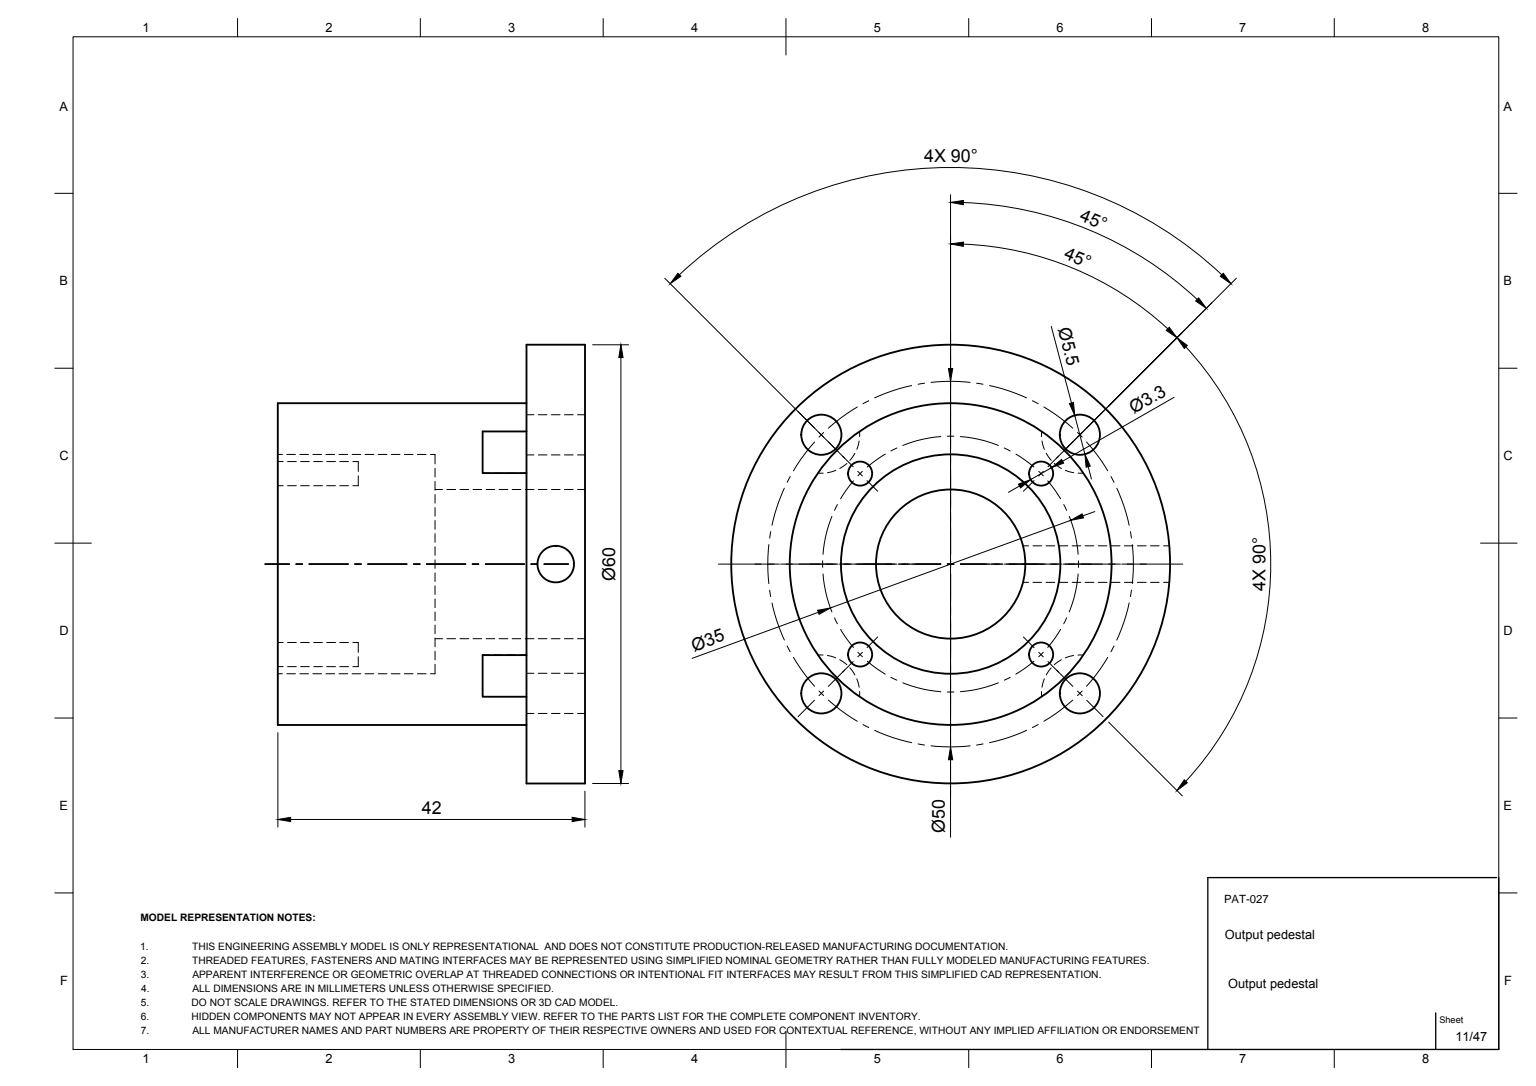
ISO-10303-21;
HEADER;
/* Generated by software containing ST-Developer
 * from STEP Tools, Inc. (www.steptools.com) 
 */

FILE_DESCRIPTION(
/* description */ ('Crank-driven oscillating fan base (mechanism only)'),

/* implementation_level */ '2;1');

FILE_NAME(
/* name */ 'Output pedestal.step',
/* time_stamp */ '2026-10-28T03:25:00-07:00',
/* author */ (''),
/* organization */ (''),
/* preprocessor_version */ 'ST-DEVELOPER v20.2',
/* originating_system */ 'Autodesk Translation Framework v15.17.0.0',
/* authorisation */ '');

FILE_SCHEMA (('AUTOMOTIVE_DESIGN { 1 0 10303 214 3 1 1 }'));
ENDSEC;

DATA;
#10=MECHANICAL_DESIGN_GEOMETRIC_PRESENTATION_REPRESENTATION('',(#443),#11916);
#320=B_SPLINE_CURVE_WITH_KNOTS('',3,(#9944,#9945,#9946,#9947,#9948,#9949,
#9950,#9951,#9952,#9953),.UNSPECIFIED.,.F.,.F.,(4,2,2,2,4),(0.,0.094594182476448,
0.189188364952896,0.283770357603024,0.378352350253152),.UNSPECIFIED.);
#321=B_SPLINE_CURVE_WITH_KNOTS('',3,(#9954,#9955,#9956,#9957,#9958,#9959,
#9960,#9961,#9962,#9963,#9964,#9965,#9966,#9967,#9968,#9969,#9970,#9971,
#9972,#9973,#9974,#9975,#9976,#9977,#9978,#9979),.UNSPECIFIED.,.F.,.F.,
(4,2,2,2,2,2,2,2,2,2,2,2,4),(0.378352350253152,0.47293434290328,0.567516335553408,
0.662110518029856,0.756704700506304,0.851298882982751,0.945893065459199,
1.04047505810933,1.13505705075946,1.22963904340958,1.32422103605971,1.41881521853616,
1.51340940101261),.UNSPECIFIED.);
#322=B_SPLINE_CURVE_WITH_KNOTS('',3,(#9983,#9984,#9985,#9986,#9987,#9988,
#9989,#9990,#9991,#9992,#9993,#9994,#9995,#9996,#9997,#9998,#9999,#10000,
#10001,#10002,#10003,#10004,#10005,#10006,#10007,#10008),.UNSPECIFIED.,
 .F.,.F.,(4,2,2,2,2,2,2,2,2,2,2,2,4),(0.,0.0942186410044058,0.188437282008812,
0.282655768798837,0.376874255588861,0.471092742378886,0.565311229168911,
0.659529870173317,0.753748511177723,0.847967152182129,0.942185793186535,
1.03640427997656,1.13062276676658),.UNSPECIFIED.);
#323=B_SPLINE_CURVE_WITH_KNOTS('',3,(#10009,#10010,#10011,#10012,#10013,
#10014,#10015,#10016,#10017,#10018),.UNSPECIFIED.,.F.,.F.,(4,2,2,2,4),(1.13062276676658,
1.22484125355661,1.31905974034663,1.41327838135104,1.50749702235545),
 .UNSPECIFIED.);
#363=SHAPE_REPRESENTATION_RELATIONSHIP('SRR','None',#12087,#403);
#403=ADVANCED_BREP_SHAPE_REPRESENTATION('',(#491),#11878);
#443=STYLED_ITEM('',(#12368),#491);
#491=MANIFOLD_SOLID_BREP('Body1',#6073);
#577=FACE_BOUND('',#1387,.T.);
#578=FACE_BOUND('',#1388,.T.);
#579=FACE_BOUND('',#1389,.T.);
#580=FACE_BOUND('',#1390,.T.);
#581=FACE_BOUND('',#1391,.T.);
#582=FACE_BOUND('',#1407,.T.);
#583=FACE_BOUND('',#1409,.T.);
#584=FACE_BOUND('',#1411,.T.);
#585=FACE_BOUND('',#1413,.T.);
#586=FACE_BOUND('',#1414,.T.);
#587=FACE_BOUND('',#1415,.T.);
#588=FACE_BOUND('',#1416,.T.);
#589=FACE_BOUND('',#1417,.T.);
#590=FACE_BOUND('',#1419,.T.);
#591=FACE_BOUND('',#1420,.T.);
#592=FACE_BOUND('',#1421,.T.);
#593=FACE_BOUND('',#1422,.T.);
#594=FACE_BOUND('',#1423,.T.);
#727=PLANE('',#6711);
#728=PLANE('',#6719);
#729=PLANE('',#6724);
#730=PLANE('',#6729);
#731=PLANE('',#6738);
#732=PLANE('',#6747);
#733=PLANE('',#6751);
#734=PLANE('',#6755);
#735=PLANE('',#6759);
#736=PLANE('',#6772);
#737=PLANE('',#6778);
#738=PLANE('',#6779);
#955=FACE_OUTER_BOUND('',#1377,.T.);
#956=FACE_OUTER_BOUND('',#1378,.T.);
#957=FACE_OUTER_BOUND('',#1379,.T.);
#958=FACE_OUTER_BOUND('',#1380,.T.);
#959=FACE_OUTER_BOUND('',#1381,.T.);
#960=FACE_OUTER_BOUND('',#1382,.T.);
#961=FACE_OUTER_BOUND('',#1383,.T.);
#962=FACE_OUTER_BOUND('',#1384,.T.);
#963=FACE_OUTER_BOUND('',#1385,.T.);
#964=FACE_OUTER_BOUND('',#1386,.T.);
#965=FACE_OUTER_BOUND('',#1392,.T.);
#966=FACE_OUTER_BOUND('',#1393,.T.);
#967=FACE_OUTER_BOUND('',#1394,.T.);
#968=FACE_OUTER_BOUND('',#1395,.T.);
#969=FACE_OUTER_BOUND('',#1396,.T.);
#970=FACE_OUTER_BOUND('',#1397,.T.);
#971=FACE_OUTER_BOUND('',#1398,.T.);
#972=FACE_OUTER_BOUND('',#1399,.T.);
#973=FACE_OUTER_BOUND('',#1400,.T.);
#974=FACE_OUTER_BOUND('',#1401,.T.);
#975=FACE_OUTER_BOUND('',#1402,.T.);
#976=FACE_OUTER_BOUND('',#1403,.T.);
#977=FACE_OUTER_BOUND('',#1404,.T.);
#978=FACE_OUTER_BOUND('',#1405,.T.);
#979=FACE_OUTER_BOUND('',#1406,.T.);
#980=FACE_OUTER_BOUND('',#1408,.T.);
#981=FACE_OUTER_BOUND('',#1410,.T.);
#982=FACE_OUTER_BOUND('',#1412,.T.);
#983=FACE_OUTER_BOUND('',#1418,.T.);
#1377=EDGE_LOOP('',(#4372,#4373));
#1378=EDGE_LOOP('',(#4374,#4375,#4376,#4377));
#1379=EDGE_LOOP('',(#4378,#4379,#4380,#4381));
#1380=EDGE_LOOP('',(#4382,#4383));
#1381=EDGE_LOOP('',(#4384,#4385,#4386,#4387));
#1382=EDGE_LOOP('',(#4388,#4389));
#1383=EDGE_LOOP('',(#4390,#4391,#4392,#4393));
#1384=EDGE_LOOP('',(#4394,#4395));
#1385=EDGE_LOOP('',(#4396,#4397,#4398,#4399,#4400,#4401,#4402,#4403,#4404,
#4405,#4406,#4407,#4408,#4409,#4410,#4411,#4412,#4413,#4414,#4415));
#1386=EDGE_LOOP('',(#4416));
#1387=EDGE_LOOP('',(#4417,#4418,#4419,#4420,#4421,#4422,#4423,#4424,#4425));
#1388=EDGE_LOOP('',(#4426));
#1389=EDGE_LOOP('',(#4427));
#1390=EDGE_LOOP('',(#4428));
#1391=EDGE_LOOP('',(#4429));
#1392=EDGE_LOOP('',(#4430,#4431,#4432,#4433));
#1393=EDGE_LOOP('',(#4434));
#1394=EDGE_LOOP('',(#4435,#4436,#4437,#4438));
#1395=EDGE_LOOP('',(#4439));
#1396=EDGE_LOOP('',(#4440,#4441,#4442,#4443));
#1397=EDGE_LOOP('',(#4444));
#1398=EDGE_LOOP('',(#4445,#4446,#4447,#4448));
#1399=EDGE_LOOP('',(#4449));
#1400=EDGE_LOOP('',(#4450,#4451,#4452,#4453,#4454,#4455));
#1401=EDGE_LOOP('',(#4456,#4457,#4458,#4459));
#1402=EDGE_LOOP('',(#4460,#4461,#4462,#4463));
#1403=EDGE_LOOP('',(#4464,#4465,#4466,#4467));
#1404=EDGE_LOOP('',(#4468,#4469,#4470,#4471));
#1405=EDGE_LOOP('',(#4472,#4473,#4474,#4475));
#1406=EDGE_LOOP('',(#4476));
#1407=EDGE_LOOP('',(#4477));
#1408=EDGE_LOOP('',(#4478,#4479,#4480,#4481));
#1409=EDGE_LOOP('',(#4482,#4483));
#1410=EDGE_LOOP('',(#4484,#4485,#4486,#4487));
#1411=EDGE_LOOP('',(#4488,#4489));
#1412=EDGE_LOOP('',(#4490));
#1413=EDGE_LOOP('',(#4491));
#1414=EDGE_LOOP('',(#4492));
#1415=EDGE_LOOP('',(#4493));
#1416=EDGE_LOOP('',(#4494));
#1417=EDGE_LOOP('',(#4495));
#1418=EDGE_LOOP('',(#4496));
#1419=EDGE_LOOP('',(#4497));
#1420=EDGE_LOOP('',(#4498));
#1421=EDGE_LOOP('',(#4499));
#1422=EDGE_LOOP('',(#4500));
#1423=EDGE_LOOP('',(#4501));
#1872=LINE('',#9855,#2205);
#1873=LINE('',#9858,#2206);
#1874=LINE('',#9862,#2207);
#1875=LINE('',#9866,#2208);
#1876=LINE('',#9873,#2209);
#1877=LINE('',#9877,#2210);
#1878=LINE('',#9884,#2211);
#1879=LINE('',#9888,#2212);
#1880=LINE('',#9896,#2213);
#1881=LINE('',#9917,#2214);
#1882=LINE('',#9924,#2215);
#1883=LINE('',#9931,#2216);
#1884=LINE('',#9938,#2217);
#1885=LINE('',#9981,#2218);
#1886=LINE('',#10022,#2219);
#1887=LINE('',#10026,#2220);
#1888=LINE('',#10030,#2221);
#1889=LINE('',#10034,#2222);
#1890=LINE('',#10039,#2223);
#1891=LINE('',#10046,#2224);
#1892=LINE('',#10050,#2225);
#2205=VECTOR('',#7797,1.);
#2206=VECTOR('',#7800,1.);
#2207=VECTOR('',#7803,1.);
#2208=VECTOR('',#7806,1.);
#2209=VECTOR('',#7815,1.);
#2210=VECTOR('',#7818,1.);
#2211=VECTOR('',#7827,1.);
#2212=VECTOR('',#7830,1.);
#2213=VECTOR('',#7841,2.2);
#2214=VECTOR('',#7868,0.165);
#2215=VECTOR('',#7877,0.165);
#2216=VECTOR('',#7886,0.164999999999999);
#2217=VECTOR('',#7895,0.164999999999999);
#2218=VECTOR('',#7902,0.25);
#2219=VECTOR('',#7907,0.275);
#2220=VECTOR('',#7912,0.275);
#2221=VECTOR('',#7917,0.275);
#2222=VECTOR('',#7922,0.275);
#2223=VECTOR('',#7927,1.5);
#2224=VECTOR('',#7936,3.);
#2225=VECTOR('',#7941,1.02);
#2538=CIRCLE('',#6712,2.2);
#2539=CIRCLE('',#6713,0.525);
#2540=CIRCLE('',#6715,0.525);
#2541=CIRCLE('',#6717,0.525);
#2542=CIRCLE('',#6718,0.525);
#2543=CIRCLE('',#6720,2.2);
#2544=CIRCLE('',#6722,0.525);
#2545=CIRCLE('',#6723,0.525);
#2546=CIRCLE('',#6725,2.2);
#2547=CIRCLE('',#6727,0.525);
#2548=CIRCLE('',#6728,0.525);
#2549=CIRCLE('',#6730,2.2);
#2550=CIRCLE('',#6732,2.2);
#2551=CIRCLE('',#6733,2.2);
#2552=CIRCLE('',#6734,2.2);
#2553=CIRCLE('',#6735,2.2);
#2554=CIRCLE('',#6736,2.2);
#2555=CIRCLE('',#6737,2.2);
#2556=CIRCLE('',#6739,3.);
#2557=CIRCLE('',#6740,0.275);
#2558=CIRCLE('',#6741,0.275);
#2559=CIRCLE('',#6742,0.275);
#2560=CIRCLE('',#6743,0.275);
#2561=CIRCLE('',#6745,0.165);
#2562=CIRCLE('',#6746,0.165);
#2563=CIRCLE('',#6749,0.165);
#2564=CIRCLE('',#6750,0.165);
#2565=CIRCLE('',#6753,0.164999999999999);
#2566=CIRCLE('',#6754,0.164999999999999);
#2567=CIRCLE('',#6757,0.164999999999999);
#2568=CIRCLE('',#6758,0.164999999999999);
#2569=CIRCLE('',#6762,0.275);
#2570=CIRCLE('',#6764,0.275);
#2571=CIRCLE('',#6766,0.275);
#2572=CIRCLE('',#6768,0.275);
#2573=CIRCLE('',#6770,1.5);
#2574=CIRCLE('',#6771,1.5);
#2575=CIRCLE('',#6773,1.02);
#2576=CIRCLE('',#6775,3.);
#2577=CIRCLE('',#6777,1.02);
#2931=VERTEX_POINT('',#9849);
#2932=VERTEX_POINT('',#9850);
#2933=VERTEX_POINT('',#9854);
#2934=VERTEX_POINT('',#9856);
#2935=VERTEX_POINT('',#9860);
#2936=VERTEX_POINT('',#9861);
#2937=VERTEX_POINT('',#9863);
#2938=VERTEX_POINT('',#9865);
#2939=VERTEX_POINT('',#9871);
#2940=VERTEX_POINT('',#9872);
#2941=VERTEX_POINT('',#9874);
#2942=VERTEX_POINT('',#9876);
#2943=VERTEX_POINT('',#9882);
#2944=VERTEX_POINT('',#9883);
#2945=VERTEX_POINT('',#9885);
#2946=VERTEX_POINT('',#9887);
#2947=VERTEX_POINT('',#9893);
#2948=VERTEX_POINT('',#9895);
#2949=VERTEX_POINT('',#9903);
#2950=VERTEX_POINT('',#9905);
#2951=VERTEX_POINT('',#9907);
#2952=VERTEX_POINT('',#9909);
#2953=VERTEX_POINT('',#9911);
#2954=VERTEX_POINT('',#9914);
#2955=VERTEX_POINT('',#9916);
#2956=VERTEX_POINT('',#9921);
#2957=VERTEX_POINT('',#9923);
#2958=VERTEX_POINT('',#9928);
#2959=VERTEX_POINT('',#9930);
#2960=VERTEX_POINT('',#9935);
#2961=VERTEX_POINT('',#9937);
#2962=VERTEX_POINT('',#9942);
#2963=VERTEX_POINT('',#9943);
#2964=VERTEX_POINT('',#9980);
#2965=VERTEX_POINT('',#9982);
#2966=VERTEX_POINT('',#10020);
#2967=VERTEX_POINT('',#10024);
#2968=VERTEX_POINT('',#10028);
#2969=VERTEX_POINT('',#10032);
#2970=VERTEX_POINT('',#10036);
#2971=VERTEX_POINT('',#10038);
#2972=VERTEX_POINT('',#10042);
#2973=VERTEX_POINT('',#10045);
#2974=VERTEX_POINT('',#10049);
#3481=EDGE_CURVE('',#2931,#2932,#2538,.T.);
#3482=EDGE_CURVE('',#2932,#2931,#2539,.T.);
#3483=EDGE_CURVE('',#2933,#2931,#1872,.T.);
#3484=EDGE_CURVE('',#2934,#2933,#2540,.T.);
#3485=EDGE_CURVE('',#2932,#2934,#1873,.T.);
#3486=EDGE_CURVE('',#2935,#2936,#1874,.T.);
#3487=EDGE_CURVE('',#2935,#2937,#2541,.T.);
#3488=EDGE_CURVE('',#2938,#2937,#1875,.T.);
#3489=EDGE_CURVE('',#2936,#2938,#2542,.T.);
#3490=EDGE_CURVE('',#2937,#2935,#2543,.T.);
#3491=EDGE_CURVE('',#2939,#2940,#1876,.T.);
#3492=EDGE_CURVE('',#2939,#2941,#2544,.T.);
#3493=EDGE_CURVE('',#2942,#2941,#1877,.T.);
#3494=EDGE_CURVE('',#2940,#2942,#2545,.T.);
#3495=EDGE_CURVE('',#2941,#2939,#2546,.T.);
#3496=EDGE_CURVE('',#2943,#2944,#1878,.T.);
#3497=EDGE_CURVE('',#2943,#2945,#2547,.T.);
#3498=EDGE_CURVE('',#2946,#2945,#1879,.T.);
#3499=EDGE_CURVE('',#2944,#2946,#2548,.T.);
#3500=EDGE_CURVE('',#2945,#2943,#2549,.T.);
#3501=EDGE_CURVE('',#2947,#2947,#2550,.T.);
#3502=EDGE_CURVE('',#2947,#2948,#1880,.T.);
#3503=EDGE_CURVE('',#2948,#2933,#2551,.T.);
#3504=EDGE_CURVE('',#2934,#2946,#2552,.T.);
#3505=EDGE_CURVE('',#2944,#2942,#2553,.T.);
#3506=EDGE_CURVE('',#2940,#2938,#2554,.T.);
#3507=EDGE_CURVE('',#2936,#2948,#2555,.T.);
#3508=EDGE_CURVE('',#2949,#2949,#2556,.T.);
#3509=EDGE_CURVE('',#2950,#2950,#2557,.T.);
#3510=EDGE_CURVE('',#2951,#2951,#2558,.T.);
#3511=EDGE_CURVE('',#2952,#2952,#2559,.T.);
#3512=EDGE_CURVE('',#2953,#2953,#2560,.T.);
#3513=EDGE_CURVE('',#2954,#2954,#2561,.T.);
#3514=EDGE_CURVE('',#2954,#2955,#1881,.T.);
#3515=EDGE_CURVE('',#2955,#2955,#2562,.T.);
#3516=EDGE_CURVE('',#2956,#2956,#2563,.T.);
#3517=EDGE_CURVE('',#2956,#2957,#1882,.T.);
#3518=EDGE_CURVE('',#2957,#2957,#2564,.T.);
#3519=EDGE_CURVE('',#2958,#2958,#2565,.T.);
#3520=EDGE_CURVE('',#2958,#2959,#1883,.T.);
#3521=EDGE_CURVE('',#2959,#2959,#2566,.T.);
#3522=EDGE_CURVE('',#2960,#2960,#2567,.T.);
#3523=EDGE_CURVE('',#2960,#2961,#1884,.T.);
#3524=EDGE_CURVE('',#2961,#2961,#2568,.T.);
#3525=EDGE_CURVE('',#2962,#2963,#320,.T.);
#3526=EDGE_CURVE('',#2963,#2962,#321,.T.);
#3527=EDGE_CURVE('',#2963,#2964,#1885,.T.);
#3528=EDGE_CURVE('',#2965,#2964,#322,.T.);
#3529=EDGE_CURVE('',#2964,#2965,#323,.T.);
#3530=EDGE_CURVE('',#2966,#2966,#2569,.T.);
#3531=EDGE_CURVE('',#2966,#2950,#1886,.T.);
#3532=EDGE_CURVE('',#2967,#2967,#2570,.T.);
#3533=EDGE_CURVE('',#2967,#2953,#1887,.T.);
#3534=EDGE_CURVE('',#2968,#2968,#2571,.T.);
#3535=EDGE_CURVE('',#2968,#2951,#1888,.T.);
#3536=EDGE_CURVE('',#2969,#2969,#2572,.T.);
#3537=EDGE_CURVE('',#2969,#2952,#1889,.T.);
#3538=EDGE_CURVE('',#2970,#2970,#2573,.T.);
#3539=EDGE_CURVE('',#2970,#2971,#1890,.T.);
#3540=EDGE_CURVE('',#2971,#2971,#2574,.T.);
#3541=EDGE_CURVE('',#2972,#2972,#2575,.T.);
#3542=EDGE_CURVE('',#2949,#2973,#1891,.T.);
#3543=EDGE_CURVE('',#2973,#2973,#2576,.T.);
#3544=EDGE_CURVE('',#2972,#2974,#1892,.T.);
#3545=EDGE_CURVE('',#2974,#2974,#2577,.T.);
#4372=ORIENTED_EDGE('',*,*,#3481,.F.);
#4373=ORIENTED_EDGE('',*,*,#3482,.F.);
#4374=ORIENTED_EDGE('',*,*,#3483,.F.);
#4375=ORIENTED_EDGE('',*,*,#3484,.F.);
#4376=ORIENTED_EDGE('',*,*,#3485,.F.);
#4377=ORIENTED_EDGE('',*,*,#3482,.T.);
#4378=ORIENTED_EDGE('',*,*,#3486,.F.);
#4379=ORIENTED_EDGE('',*,*,#3487,.T.);
#4380=ORIENTED_EDGE('',*,*,#3488,.F.);
#4381=ORIENTED_EDGE('',*,*,#3489,.F.);
#4382=ORIENTED_EDGE('',*,*,#3490,.F.);
#4383=ORIENTED_EDGE('',*,*,#3487,.F.);
#4384=ORIENTED_EDGE('',*,*,#3491,.F.);
#4385=ORIENTED_EDGE('',*,*,#3492,.T.);
#4386=ORIENTED_EDGE('',*,*,#3493,.F.);
#4387=ORIENTED_EDGE('',*,*,#3494,.F.);
#4388=ORIENTED_EDGE('',*,*,#3495,.F.);
#4389=ORIENTED_EDGE('',*,*,#3492,.F.);
#4390=ORIENTED_EDGE('',*,*,#3496,.F.);
#4391=ORIENTED_EDGE('',*,*,#3497,.T.);
#4392=ORIENTED_EDGE('',*,*,#3498,.F.);
#4393=ORIENTED_EDGE('',*,*,#3499,.F.);
#4394=ORIENTED_EDGE('',*,*,#3500,.F.);
#4395=ORIENTED_EDGE('',*,*,#3497,.F.);
#4396=ORIENTED_EDGE('',*,*,#3501,.F.);
#4397=ORIENTED_EDGE('',*,*,#3502,.T.);
#4398=ORIENTED_EDGE('',*,*,#3503,.T.);
#4399=ORIENTED_EDGE('',*,*,#3483,.T.);
#4400=ORIENTED_EDGE('',*,*,#3481,.T.);
#4401=ORIENTED_EDGE('',*,*,#3485,.T.);
#4402=ORIENTED_EDGE('',*,*,#3504,.T.);
#4403=ORIENTED_EDGE('',*,*,#3498,.T.);
#4404=ORIENTED_EDGE('',*,*,#3500,.T.);
#4405=ORIENTED_EDGE('',*,*,#3496,.T.);
#4406=ORIENTED_EDGE('',*,*,#3505,.T.);
#4407=ORIENTED_EDGE('',*,*,#3493,.T.);
#4408=ORIENTED_EDGE('',*,*,#3495,.T.);
#4409=ORIENTED_EDGE('',*,*,#3491,.T.);
#4410=ORIENTED_EDGE('',*,*,#3506,.T.);
#4411=ORIENTED_EDGE('',*,*,#3488,.T.);
#4412=ORIENTED_EDGE('',*,*,#3490,.T.);
#4413=ORIENTED_EDGE('',*,*,#3486,.T.);
#4414=ORIENTED_EDGE('',*,*,#3507,.T.);
#4415=ORIENTED_EDGE('',*,*,#3502,.F.);
#4416=ORIENTED_EDGE('',*,*,#3508,.T.);
#4417=ORIENTED_EDGE('',*,*,#3507,.F.);
#4418=ORIENTED_EDGE('',*,*,#3489,.T.);
#4419=ORIENTED_EDGE('',*,*,#3506,.F.);
#4420=ORIENTED_EDGE('',*,*,#3494,.T.);
#4421=ORIENTED_EDGE('',*,*,#3505,.F.);
#4422=ORIENTED_EDGE('',*,*,#3499,.T.);
#4423=ORIENTED_EDGE('',*,*,#3504,.F.);
#4424=ORIENTED_EDGE('',*,*,#3484,.T.);
#4425=ORIENTED_EDGE('',*,*,#3503,.F.);
#4426=ORIENTED_EDGE('',*,*,#3509,.T.);
#4427=ORIENTED_EDGE('',*,*,#3510,.T.);
#4428=ORIENTED_EDGE('',*,*,#3511,.T.);
#4429=ORIENTED_EDGE('',*,*,#3512,.T.);
#4430=ORIENTED_EDGE('',*,*,#3513,.F.);
#4431=ORIENTED_EDGE('',*,*,#3514,.T.);
#4432=ORIENTED_EDGE('',*,*,#3515,.F.);
#4433=ORIENTED_EDGE('',*,*,#3514,.F.);
#4434=ORIENTED_EDGE('',*,*,#3513,.T.);
#4435=ORIENTED_EDGE('',*,*,#3516,.F.);
#4436=ORIENTED_EDGE('',*,*,#3517,.T.);
#4437=ORIENTED_EDGE('',*,*,#3518,.F.);
#4438=ORIENTED_EDGE('',*,*,#3517,.F.);
#4439=ORIENTED_EDGE('',*,*,#3516,.T.);
#4440=ORIENTED_EDGE('',*,*,#3519,.F.);
#4441=ORIENTED_EDGE('',*,*,#3520,.T.);
#4442=ORIENTED_EDGE('',*,*,#3521,.F.);
#4443=ORIENTED_EDGE('',*,*,#3520,.F.);
#4444=ORIENTED_EDGE('',*,*,#3519,.T.);
#4445=ORIENTED_EDGE('',*,*,#3522,.F.);
#4446=ORIENTED_EDGE('',*,*,#3523,.T.);
#4447=ORIENTED_EDGE('',*,*,#3524,.F.);
#4448=ORIENTED_EDGE('',*,*,#3523,.F.);
#4449=ORIENTED_EDGE('',*,*,#3522,.T.);
#4450=ORIENTED_EDGE('',*,*,#3525,.F.);
#4451=ORIENTED_EDGE('',*,*,#3526,.F.);
#4452=ORIENTED_EDGE('',*,*,#3527,.T.);
#4453=ORIENTED_EDGE('',*,*,#3528,.F.);
#4454=ORIENTED_EDGE('',*,*,#3529,.F.);
#4455=ORIENTED_EDGE('',*,*,#3527,.F.);
#4456=ORIENTED_EDGE('',*,*,#3530,.F.);
#4457=ORIENTED_EDGE('',*,*,#3531,.T.);
#4458=ORIENTED_EDGE('',*,*,#3509,.F.);
#4459=ORIENTED_EDGE('',*,*,#3531,.F.);
#4460=ORIENTED_EDGE('',*,*,#3532,.F.);
#4461=ORIENTED_EDGE('',*,*,#3533,.T.);
#4462=ORIENTED_EDGE('',*,*,#3512,.F.);
#4463=ORIENTED_EDGE('',*,*,#3533,.F.);
#4464=ORIENTED_EDGE('',*,*,#3534,.F.);
#4465=ORIENTED_EDGE('',*,*,#3535,.T.);
#4466=ORIENTED_EDGE('',*,*,#3510,.F.);
#4467=ORIENTED_EDGE('',*,*,#3535,.F.);
#4468=ORIENTED_EDGE('',*,*,#3536,.F.);
#4469=ORIENTED_EDGE('',*,*,#3537,.T.);
#4470=ORIENTED_EDGE('',*,*,#3511,.F.);
#4471=ORIENTED_EDGE('',*,*,#3537,.F.);
#4472=ORIENTED_EDGE('',*,*,#3538,.F.);
#4473=ORIENTED_EDGE('',*,*,#3539,.T.);
#4474=ORIENTED_EDGE('',*,*,#3540,.F.);
#4475=ORIENTED_EDGE('',*,*,#3539,.F.);
#4476=ORIENTED_EDGE('',*,*,#3538,.T.);
#4477=ORIENTED_EDGE('',*,*,#3541,.F.);
#4478=ORIENTED_EDGE('',*,*,#3508,.F.);
#4479=ORIENTED_EDGE('',*,*,#3542,.T.);
#4480=ORIENTED_EDGE('',*,*,#3543,.T.);
#4481=ORIENTED_EDGE('',*,*,#3542,.F.);
#4482=ORIENTED_EDGE('',*,*,#3528,.T.);
#4483=ORIENTED_EDGE('',*,*,#3529,.T.);
#4484=ORIENTED_EDGE('',*,*,#3541,.T.);
#4485=ORIENTED_EDGE('',*,*,#3544,.T.);
#4486=ORIENTED_EDGE('',*,*,#3545,.T.);
#4487=ORIENTED_EDGE('',*,*,#3544,.F.);
#4488=ORIENTED_EDGE('',*,*,#3525,.T.);
#4489=ORIENTED_EDGE('',*,*,#3526,.T.);
#4490=ORIENTED_EDGE('',*,*,#3501,.T.);
#4491=ORIENTED_EDGE('',*,*,#3540,.T.);
#4492=ORIENTED_EDGE('',*,*,#3524,.T.);
#4493=ORIENTED_EDGE('',*,*,#3521,.T.);
#4494=ORIENTED_EDGE('',*,*,#3518,.T.);
#4495=ORIENTED_EDGE('',*,*,#3515,.T.);
#4496=ORIENTED_EDGE('',*,*,#3543,.F.);
#4497=ORIENTED_EDGE('',*,*,#3545,.F.);
#4498=ORIENTED_EDGE('',*,*,#3536,.T.);
#4499=ORIENTED_EDGE('',*,*,#3534,.T.);
#4500=ORIENTED_EDGE('',*,*,#3532,.T.);
#4501=ORIENTED_EDGE('',*,*,#3530,.T.);
#5580=CYLINDRICAL_SURFACE('',#6714,0.525);
#5581=CYLINDRICAL_SURFACE('',#6716,0.525);
#5582=CYLINDRICAL_SURFACE('',#6721,0.525);
#5583=CYLINDRICAL_SURFACE('',#6726,0.525);
#5584=CYLINDRICAL_SURFACE('',#6731,2.2);
#5585=CYLINDRICAL_SURFACE('',#6744,0.165);
#5586=CYLINDRICAL_SURFACE('',#6748,0.165);
#5587=CYLINDRICAL_SURFACE('',#6752,0.164999999999999);
#5588=CYLINDRICAL_SURFACE('',#6756,0.164999999999999);
#5589=CYLINDRICAL_SURFACE('',#6760,0.25);
#5590=CYLINDRICAL_SURFACE('',#6761,0.275);
#5591=CYLINDRICAL_SURFACE('',#6763,0.275);
#5592=CYLINDRICAL_SURFACE('',#6765,0.275);
#5593=CYLINDRICAL_SURFACE('',#6767,0.275);
#5594=CYLINDRICAL_SURFACE('',#6769,1.5);
#5595=CYLINDRICAL_SURFACE('',#6774,3.);
#5596=CYLINDRICAL_SURFACE('',#6776,1.02);
#5761=ADVANCED_FACE('',(#955),#727,.F.);
#5762=ADVANCED_FACE('',(#956),#5580,.F.);
#5763=ADVANCED_FACE('',(#957),#5581,.F.);
#5764=ADVANCED_FACE('',(#958),#728,.F.);
#5765=ADVANCED_FACE('',(#959),#5582,.F.);
#5766=ADVANCED_FACE('',(#960),#729,.F.);
#5767=ADVANCED_FACE('',(#961),#5583,.F.);
#5768=ADVANCED_FACE('',(#962),#730,.F.);
#5769=ADVANCED_FACE('',(#963),#5584,.T.);
#5770=ADVANCED_FACE('',(#964,#577,#578,#579,#580,#581),#731,.T.);
#5771=ADVANCED_FACE('',(#965),#5585,.F.);
#5772=ADVANCED_FACE('',(#966),#732,.T.);
#5773=ADVANCED_FACE('',(#967),#5586,.F.);
#5774=ADVANCED_FACE('',(#968),#733,.T.);
#5775=ADVANCED_FACE('',(#969),#5587,.F.);
#5776=ADVANCED_FACE('',(#970),#734,.T.);
#5777=ADVANCED_FACE('',(#971),#5588,.F.);
#5778=ADVANCED_FACE('',(#972),#735,.T.);
#5779=ADVANCED_FACE('',(#973),#5589,.F.);
#5780=ADVANCED_FACE('',(#974),#5590,.F.);
#5781=ADVANCED_FACE('',(#975),#5591,.F.);
#5782=ADVANCED_FACE('',(#976),#5592,.F.);
#5783=ADVANCED_FACE('',(#977),#5593,.F.);
#5784=ADVANCED_FACE('',(#978),#5594,.F.);
#5785=ADVANCED_FACE('',(#979,#582),#736,.T.);
#5786=ADVANCED_FACE('',(#980,#583),#5595,.T.);
#5787=ADVANCED_FACE('',(#981,#584),#5596,.F.);
#5788=ADVANCED_FACE('',(#982,#585,#586,#587,#588,#589),#737,.T.);
#5789=ADVANCED_FACE('',(#983,#590,#591,#592,#593,#594),#738,.F.);
#6073=CLOSED_SHELL('',(#5761,#5762,#5763,#5764,#5765,#5766,#5767,#5768,
#5769,#5770,#5771,#5772,#5773,#5774,#5775,#5776,#5777,#5778,#5779,#5780,
#5781,#5782,#5783,#5784,#5785,#5786,#5787,#5788,#5789));
#6710=AXIS2_PLACEMENT_3D('',#9847,#7787,#7788);
#6711=AXIS2_PLACEMENT_3D('',#9848,#7789,#7790);
#6712=AXIS2_PLACEMENT_3D('',#9851,#7791,#7792);
#6713=AXIS2_PLACEMENT_3D('',#9852,#7793,#7794);
#6714=AXIS2_PLACEMENT_3D('',#9853,#7795,#7796);
#6715=AXIS2_PLACEMENT_3D('',#9857,#7798,#7799);
#6716=AXIS2_PLACEMENT_3D('',#9859,#7801,#7802);
#6717=AXIS2_PLACEMENT_3D('',#9864,#7804,#7805);
#6718=AXIS2_PLACEMENT_3D('',#9867,#7807,#7808);
#6719=AXIS2_PLACEMENT_3D('',#9868,#7809,#7810);
#6720=AXIS2_PLACEMENT_3D('',#9869,#7811,#7812);
#6721=AXIS2_PLACEMENT_3D('',#9870,#7813,#7814);
#6722=AXIS2_PLACEMENT_3D('',#9875,#7816,#7817);
#6723=AXIS2_PLACEMENT_3D('',#9878,#7819,#7820);
#6724=AXIS2_PLACEMENT_3D('',#9879,#7821,#7822);
#6725=AXIS2_PLACEMENT_3D('',#9880,#7823,#7824);
#6726=AXIS2_PLACEMENT_3D('',#9881,#7825,#7826);
#6727=AXIS2_PLACEMENT_3D('',#9886,#7828,#7829);
#6728=AXIS2_PLACEMENT_3D('',#9889,#7831,#7832);
#6729=AXIS2_PLACEMENT_3D('',#9890,#7833,#7834);
#6730=AXIS2_PLACEMENT_3D('',#9891,#7835,#7836);
#6731=AXIS2_PLACEMENT_3D('',#9892,#7837,#7838);
#6732=AXIS2_PLACEMENT_3D('',#9894,#7839,#7840);
#6733=AXIS2_PLACEMENT_3D('',#9897,#7842,#7843);
#6734=AXIS2_PLACEMENT_3D('',#9898,#7844,#7845);
#6735=AXIS2_PLACEMENT_3D('',#9899,#7846,#7847);
#6736=AXIS2_PLACEMENT_3D('',#9900,#7848,#7849);
#6737=AXIS2_PLACEMENT_3D('',#9901,#7850,#7851);
#6738=AXIS2_PLACEMENT_3D('',#9902,#7852,#7853);
#6739=AXIS2_PLACEMENT_3D('',#9904,#7854,#7855);
#6740=AXIS2_PLACEMENT_3D('',#9906,#7856,#7857);
#6741=AXIS2_PLACEMENT_3D('',#9908,#7858,#7859);
#6742=AXIS2_PLACEMENT_3D('',#9910,#7860,#7861);
#6743=AXIS2_PLACEMENT_3D('',#9912,#7862,#7863);
#6744=AXIS2_PLACEMENT_3D('',#9913,#7864,#7865);
#6745=AXIS2_PLACEMENT_3D('',#9915,#7866,#7867);
#6746=AXIS2_PLACEMENT_3D('',#9918,#7869,#7870);
#6747=AXIS2_PLACEMENT_3D('',#9919,#7871,#7872);
#6748=AXIS2_PLACEMENT_3D('',#9920,#7873,#7874);
#6749=AXIS2_PLACEMENT_3D('',#9922,#7875,#7876);
#6750=AXIS2_PLACEMENT_3D('',#9925,#7878,#7879);
#6751=AXIS2_PLACEMENT_3D('',#9926,#7880,#7881);
#6752=AXIS2_PLACEMENT_3D('',#9927,#7882,#7883);
#6753=AXIS2_PLACEMENT_3D('',#9929,#7884,#7885);
#6754=AXIS2_PLACEMENT_3D('',#9932,#7887,#7888);
#6755=AXIS2_PLACEMENT_3D('',#9933,#7889,#7890);
#6756=AXIS2_PLACEMENT_3D('',#9934,#7891,#7892);
#6757=AXIS2_PLACEMENT_3D('',#9936,#7893,#7894);
#6758=AXIS2_PLACEMENT_3D('',#9939,#7896,#7897);
#6759=AXIS2_PLACEMENT_3D('',#9940,#7898,#7899);
#6760=AXIS2_PLACEMENT_3D('',#9941,#7900,#7901);
#6761=AXIS2_PLACEMENT_3D('',#10019,#7903,#7904);
#6762=AXIS2_PLACEMENT_3D('',#10021,#7905,#7906);
#6763=AXIS2_PLACEMENT_3D('',#10023,#7908,#7909);
#6764=AXIS2_PLACEMENT_3D('',#10025,#7910,#7911);
#6765=AXIS2_PLACEMENT_3D('',#10027,#7913,#7914);
#6766=AXIS2_PLACEMENT_3D('',#10029,#7915,#7916);
#6767=AXIS2_PLACEMENT_3D('',#10031,#7918,#7919);
#6768=AXIS2_PLACEMENT_3D('',#10033,#7920,#7921);
#6769=AXIS2_PLACEMENT_3D('',#10035,#7923,#7924);
#6770=AXIS2_PLACEMENT_3D('',#10037,#7925,#7926);
#6771=AXIS2_PLACEMENT_3D('',#10040,#7928,#7929);
#6772=AXIS2_PLACEMENT_3D('',#10041,#7930,#7931);
#6773=AXIS2_PLACEMENT_3D('',#10043,#7932,#7933);
#6774=AXIS2_PLACEMENT_3D('',#10044,#7934,#7935);
#6775=AXIS2_PLACEMENT_3D('',#10047,#7937,#7938);
#6776=AXIS2_PLACEMENT_3D('',#10048,#7939,#7940);
#6777=AXIS2_PLACEMENT_3D('',#10051,#7942,#7943);
#6778=AXIS2_PLACEMENT_3D('',#10052,#7944,#7945);
#6779=AXIS2_PLACEMENT_3D('',#10053,#7946,#7947);
#7787=DIRECTION('axis',(0.,0.,1.));
#7788=DIRECTION('refdir',(1.,0.,0.));
#7789=DIRECTION('center_axis',(0.,0.,1.));
#7790=DIRECTION('ref_axis',(1.,0.,0.));
#7791=DIRECTION('center_axis',(0.,0.,1.));
#7792=DIRECTION('ref_axis',(1.,0.,0.));
#7793=DIRECTION('center_axis',(0.,0.,1.));
#7794=DIRECTION('ref_axis',(1.,0.,0.));
#7795=DIRECTION('center_axis',(0.,0.,1.));
#7796=DIRECTION('ref_axis',(1.,0.,0.));
#7797=DIRECTION('',(0.,0.,1.));
#7798=DIRECTION('center_axis',(0.,0.,1.));
#7799=DIRECTION('ref_axis',(1.,0.,0.));
#7800=DIRECTION('',(0.,0.,-1.));
#7801=DIRECTION('center_axis',(0.,0.,1.));
#7802=DIRECTION('ref_axis',(1.,0.,0.));
#7803=DIRECTION('',(0.,0.,-1.));
#7804=DIRECTION('center_axis',(0.,0.,1.));
#7805=DIRECTION('ref_axis',(1.,0.,0.));
#7806=DIRECTION('',(0.,0.,1.));
#7807=DIRECTION('center_axis',(0.,0.,1.));
#7808=DIRECTION('ref_axis',(1.,0.,0.));
#7809=DIRECTION('center_axis',(0.,0.,1.));
#7810=DIRECTION('ref_axis',(1.,0.,0.));
#7811=DIRECTION('center_axis',(0.,0.,1.));
#7812=DIRECTION('ref_axis',(1.,0.,0.));
#7813=DIRECTION('center_axis',(0.,0.,1.));
#7814=DIRECTION('ref_axis',(-0.707106781186546,-0.707106781186549,0.));
#7815=DIRECTION('',(0.,0.,-1.));
#7816=DIRECTION('center_axis',(0.,0.,1.));
#7817=DIRECTION('ref_axis',(1.,0.,0.));
#7818=DIRECTION('',(0.,0.,1.));
#7819=DIRECTION('center_axis',(0.,0.,1.));
#7820=DIRECTION('ref_axis',(1.,0.,0.));
#7821=DIRECTION('center_axis',(0.,0.,1.));
#7822=DIRECTION('ref_axis',(1.,0.,0.));
#7823=DIRECTION('center_axis',(0.,0.,1.));
#7824=DIRECTION('ref_axis',(1.,0.,0.));
#7825=DIRECTION('center_axis',(0.,0.,1.));
#7826=DIRECTION('ref_axis',(-0.707106781186547,0.707106781186548,0.));
#7827=DIRECTION('',(0.,0.,-1.));
#7828=DIRECTION('center_axis',(0.,0.,1.));
#7829=DIRECTION('ref_axis',(1.,0.,0.));
#7830=DIRECTION('',(0.,0.,1.));
#7831=DIRECTION('center_axis',(0.,0.,1.));
#7832=DIRECTION('ref_axis',(1.,0.,0.));
#7833=DIRECTION('center_axis',(0.,0.,1.));
#7834=DIRECTION('ref_axis',(1.,0.,0.));
#7835=DIRECTION('center_axis',(0.,0.,1.));
#7836=DIRECTION('ref_axis',(1.,0.,0.));
#7837=DIRECTION('center_axis',(0.,0.,1.));
#7838=DIRECTION('ref_axis',(1.,0.,0.));
#7839=DIRECTION('center_axis',(0.,0.,1.));
#7840=DIRECTION('ref_axis',(1.,0.,0.));
#7841=DIRECTION('',(0.,0.,-1.));
#7842=DIRECTION('center_axis',(0.,0.,1.));
#7843=DIRECTION('ref_axis',(1.,0.,0.));
#7844=DIRECTION('center_axis',(0.,0.,1.));
#7845=DIRECTION('ref_axis',(1.,0.,0.));
#7846=DIRECTION('center_axis',(0.,0.,1.));
#7847=DIRECTION('ref_axis',(1.,0.,0.));
#7848=DIRECTION('center_axis',(0.,0.,1.));
#7849=DIRECTION('ref_axis',(1.,0.,0.));
#7850=DIRECTION('center_axis',(0.,0.,1.));
#7851=DIRECTION('ref_axis',(1.,0.,0.));
#7852=DIRECTION('center_axis',(0.,0.,1.));
#7853=DIRECTION('ref_axis',(1.,0.,0.));
#7854=DIRECTION('center_axis',(0.,0.,1.));
#7855=DIRECTION('ref_axis',(1.,0.,0.));
#7856=DIRECTION('center_axis',(0.,0.,-1.));
#7857=DIRECTION('ref_axis',(1.,0.,0.));
#7858=DIRECTION('center_axis',(0.,0.,-1.));
#7859=DIRECTION('ref_axis',(1.,0.,0.));
#7860=DIRECTION('center_axis',(0.,0.,-1.));
#7861=DIRECTION('ref_axis',(1.,0.,0.));
#7862=DIRECTION('center_axis',(0.,0.,-1.));
#7863=DIRECTION('ref_axis',(1.,0.,0.));
#7864=DIRECTION('center_axis',(0.,0.,1.));
#7865=DIRECTION('ref_axis',(1.,0.,0.));
#7866=DIRECTION('center_axis',(0.,0.,1.));
#7867=DIRECTION('ref_axis',(1.,0.,0.));
#7868=DIRECTION('',(0.,0.,1.));
#7869=DIRECTION('center_axis',(0.,0.,-1.));
#7870=DIRECTION('ref_axis',(1.,0.,0.));
#7871=DIRECTION('center_axis',(0.,0.,1.));
#7872=DIRECTION('ref_axis',(1.,0.,0.));
#7873=DIRECTION('center_axis',(0.,0.,1.));
#7874=DIRECTION('ref_axis',(1.,0.,0.));
#7875=DIRECTION('center_axis',(0.,0.,1.));
#7876=DIRECTION('ref_axis',(1.,0.,0.));
#7877=DIRECTION('',(0.,0.,1.));
#7878=DIRECTION('center_axis',(0.,0.,-1.));
#7879=DIRECTION('ref_axis',(1.,0.,0.));
#7880=DIRECTION('center_axis',(0.,0.,1.));
#7881=DIRECTION('ref_axis',(1.,0.,0.));
#7882=DIRECTION('center_axis',(0.,0.,1.));
#7883=DIRECTION('ref_axis',(1.,0.,0.));
#7884=DIRECTION('center_axis',(0.,0.,1.));
#7885=DIRECTION('ref_axis',(1.,0.,0.));
#7886=DIRECTION('',(0.,0.,1.));
#7887=DIRECTION('center_axis',(0.,0.,-1.));
#7888=DIRECTION('ref_axis',(1.,0.,0.));
#7889=DIRECTION('center_axis',(0.,0.,1.));
#7890=DIRECTION('ref_axis',(1.,0.,0.));
#7891=DIRECTION('center_axis',(0.,0.,1.));
#7892=DIRECTION('ref_axis',(1.,0.,0.));
#7893=DIRECTION('center_axis',(0.,0.,1.));
#7894=DIRECTION('ref_axis',(1.,0.,0.));
#7895=DIRECTION('',(0.,0.,1.));
#7896=DIRECTION('center_axis',(0.,0.,-1.));
#7897=DIRECTION('ref_axis',(1.,0.,0.));
#7898=DIRECTION('center_axis',(0.,0.,1.));
#7899=DIRECTION('ref_axis',(1.,0.,0.));
#7900=DIRECTION('center_axis',(1.,0.,0.));
#7901=DIRECTION('ref_axis',(0.,0.,-1.));
#7902=DIRECTION('',(1.,0.,0.));
#7903=DIRECTION('center_axis',(0.,0.,1.));
#7904=DIRECTION('ref_axis',(1.,0.,0.));
#7905=DIRECTION('center_axis',(0.,0.,1.));
#7906=DIRECTION('ref_axis',(1.,0.,0.));
#7907=DIRECTION('',(0.,0.,1.));
#7908=DIRECTION('center_axis',(0.,0.,1.));
#7909=DIRECTION('ref_axis',(1.,0.,0.));
#7910=DIRECTION('center_axis',(0.,0.,1.));
#7911=DIRECTION('ref_axis',(1.,0.,0.));
#7912=DIRECTION('',(0.,0.,1.));
#7913=DIRECTION('center_axis',(0.,0.,1.));
#7914=DIRECTION('ref_axis',(1.,0.,0.));
#7915=DIRECTION('center_axis',(0.,0.,1.));
#7916=DIRECTION('ref_axis',(1.,0.,0.));
#7917=DIRECTION('',(0.,0.,1.));
#7918=DIRECTION('center_axis',(0.,0.,1.));
#7919=DIRECTION('ref_axis',(1.,0.,0.));
#7920=DIRECTION('center_axis',(0.,0.,1.));
#7921=DIRECTION('ref_axis',(1.,0.,0.));
#7922=DIRECTION('',(0.,0.,1.));
#7923=DIRECTION('center_axis',(0.,0.,1.));
#7924=DIRECTION('ref_axis',(1.,0.,0.));
#7925=DIRECTION('center_axis',(0.,0.,1.));
#7926=DIRECTION('ref_axis',(1.,0.,0.));
#7927=DIRECTION('',(0.,0.,1.));
#7928=DIRECTION('center_axis',(0.,0.,-1.));
#7929=DIRECTION('ref_axis',(1.,0.,0.));
#7930=DIRECTION('center_axis',(0.,0.,1.));
#7931=DIRECTION('ref_axis',(1.,0.,0.));
#7932=DIRECTION('center_axis',(0.,0.,1.));
#7933=DIRECTION('ref_axis',(1.,0.,0.));
#7934=DIRECTION('center_axis',(0.,0.,1.));
#7935=DIRECTION('ref_axis',(1.,0.,0.));
#7936=DIRECTION('',(0.,0.,-1.));
#7937=DIRECTION('center_axis',(0.,0.,1.));
#7938=DIRECTION('ref_axis',(1.,0.,0.));
#7939=DIRECTION('center_axis',(0.,0.,1.));
#7940=DIRECTION('ref_axis',(1.,0.,0.));
#7941=DIRECTION('',(0.,0.,-1.));
#7942=DIRECTION('center_axis',(0.,0.,-1.));
#7943=DIRECTION('ref_axis',(1.,0.,0.));
#7944=DIRECTION('center_axis',(0.,0.,1.));
#7945=DIRECTION('ref_axis',(1.,0.,0.));
#7946=DIRECTION('center_axis',(0.,0.,1.));
#7947=DIRECTION('ref_axis',(1.,0.,0.));
#9847=CARTESIAN_POINT('',(0.,0.,0.));
#9848=CARTESIAN_POINT('Origin',(6.23223304703363,-1.76776695296637,2.4));
#9849=CARTESIAN_POINT('',(6.18603626112981,-1.24480341984751,2.4));
#9850=CARTESIAN_POINT('',(6.75519658015249,-1.81396373887019,2.4));
#9851=CARTESIAN_POINT('Origin',(8.,0.,2.4));
#9852=CARTESIAN_POINT('Origin',(6.23223304703363,-1.76776695296637,2.4));
#9853=CARTESIAN_POINT('Origin',(6.23223304703363,-1.76776695296637,1.8));
#9854=CARTESIAN_POINT('',(6.18603626112981,-1.24480341984751,1.8));
#9855=CARTESIAN_POINT('',(6.18603626112981,-1.24480341984751,1.8));
#9856=CARTESIAN_POINT('',(6.75519658015249,-1.81396373887019,1.8));
#9857=CARTESIAN_POINT('Origin',(6.23223304703363,-1.76776695296637,1.8));
#9858=CARTESIAN_POINT('',(6.75519658015249,-1.81396373887019,1.8));
#9859=CARTESIAN_POINT('Origin',(6.23223304703363,1.76776695296637,1.8));
#9860=CARTESIAN_POINT('',(6.18603626112981,1.24480341984751,2.4));
#9861=CARTESIAN_POINT('',(6.18603626112981,1.24480341984751,1.8));
#9862=CARTESIAN_POINT('',(6.18603626112981,1.24480341984751,1.8));
#9863=CARTESIAN_POINT('',(6.75519658015249,1.81396373887019,2.4));
#9864=CARTESIAN_POINT('Origin',(6.23223304703363,1.76776695296637,2.4));
#9865=CARTESIAN_POINT('',(6.75519658015249,1.81396373887019,1.8));
#9866=CARTESIAN_POINT('',(6.75519658015249,1.81396373887019,1.8));
#9867=CARTESIAN_POINT('Origin',(6.23223304703363,1.76776695296637,1.8));
#9868=CARTESIAN_POINT('Origin',(6.23223304703363,1.76776695296637,2.4));
#9869=CARTESIAN_POINT('Origin',(8.,0.,2.4));
#9870=CARTESIAN_POINT('Origin',(9.76776695296637,1.76776695296637,1.8));
#9871=CARTESIAN_POINT('',(9.24480341984751,1.81396373887019,2.4));
#9872=CARTESIAN_POINT('',(9.24480341984751,1.81396373887019,1.8));
#9873=CARTESIAN_POINT('',(9.24480341984751,1.81396373887019,1.8));
#9874=CARTESIAN_POINT('',(9.8139637388702,1.24480341984751,2.4));
#9875=CARTESIAN_POINT('Origin',(9.76776695296637,1.76776695296637,2.4));
#9876=CARTESIAN_POINT('',(9.81396373887019,1.24480341984751,1.8));
#9877=CARTESIAN_POINT('',(9.8139637388702,1.24480341984751,1.8));
#9878=CARTESIAN_POINT('Origin',(9.76776695296637,1.76776695296637,1.8));
#9879=CARTESIAN_POINT('Origin',(9.76776695296637,1.76776695296637,2.4));
#9880=CARTESIAN_POINT('Origin',(8.,0.,2.4));
#9881=CARTESIAN_POINT('Origin',(9.76776695296637,-1.76776695296637,1.8));
#9882=CARTESIAN_POINT('',(9.81396373887019,-1.24480341984751,2.4));
#9883=CARTESIAN_POINT('',(9.81396373887019,-1.24480341984751,1.8));
#9884=CARTESIAN_POINT('',(9.81396373887019,-1.24480341984751,1.8));
#9885=CARTESIAN_POINT('',(9.24480341984751,-1.81396373887019,2.4));
#9886=CARTESIAN_POINT('Origin',(9.76776695296637,-1.76776695296637,2.4));
#9887=CARTESIAN_POINT('',(9.24480341984751,-1.81396373887019,1.8));
#9888=CARTESIAN_POINT('',(9.24480341984751,-1.81396373887019,1.8));
#9889=CARTESIAN_POINT('Origin',(9.76776695296637,-1.76776695296637,1.8));
#9890=CARTESIAN_POINT('Origin',(9.76776695296637,-1.76776695296637,2.4));
#9891=CARTESIAN_POINT('Origin',(8.,0.,2.4));
#9892=CARTESIAN_POINT('Origin',(8.,0.,1.));
#9893=CARTESIAN_POINT('',(5.8,-2.69422295812418E-16,5.2));
#9894=CARTESIAN_POINT('Origin',(8.,0.,5.2));
#9895=CARTESIAN_POINT('',(5.8,-2.69422295812418E-16,1.8));
#9896=CARTESIAN_POINT('',(5.8,-2.69422295812418E-16,1.));
#9897=CARTESIAN_POINT('Origin',(8.,0.,1.8));
#9898=CARTESIAN_POINT('Origin',(8.,0.,1.8));
#9899=CARTESIAN_POINT('Origin',(8.,0.,1.8));
#9900=CARTESIAN_POINT('Origin',(8.,0.,1.8));
#9901=CARTESIAN_POINT('Origin',(8.,0.,1.8));
#9902=CARTESIAN_POINT('Origin',(8.,0.,1.8));
#9903=CARTESIAN_POINT('',(5.,-3.67394039744206E-16,1.8));
#9904=CARTESIAN_POINT('Origin',(8.,0.,1.8));
#9905=CARTESIAN_POINT('',(5.95723304703363,-1.76776695296637,1.8));
#9906=CARTESIAN_POINT('Origin',(6.23223304703363,-1.76776695296637,1.8));
#9907=CARTESIAN_POINT('',(9.49276695296637,1.76776695296637,1.8));
#9908=CARTESIAN_POINT('Origin',(9.76776695296637,1.76776695296637,1.8));
#9909=CARTESIAN_POINT('',(9.49276695296637,-1.76776695296637,1.8));
#9910=CARTESIAN_POINT('Origin',(9.76776695296637,-1.76776695296637,1.8));
#9911=CARTESIAN_POINT('',(5.95723304703363,1.76776695296637,1.8));
#9912=CARTESIAN_POINT('Origin',(6.23223304703363,1.76776695296637,1.8));
#9913=CARTESIAN_POINT('Origin',(6.76256313292354,-1.23743686707646,4.1));
#9914=CARTESIAN_POINT('',(6.59756313292354,-1.23743686707646,4.1));
#9915=CARTESIAN_POINT('Origin',(6.76256313292354,-1.23743686707646,4.1));
#9916=CARTESIAN_POINT('',(6.59756313292354,-1.23743686707646,5.2));
#9917=CARTESIAN_POINT('',(6.59756313292354,-1.23743686707646,4.1));
#9918=CARTESIAN_POINT('Origin',(6.76256313292354,-1.23743686707646,5.2));
#9919=CARTESIAN_POINT('Origin',(6.76256313292354,-1.23743686707646,4.1));
#9920=CARTESIAN_POINT('Origin',(6.76256313292354,1.23743686707646,4.1));
#9921=CARTESIAN_POINT('',(6.59756313292354,1.23743686707646,4.1));
#9922=CARTESIAN_POINT('Origin',(6.76256313292354,1.23743686707646,4.1));
#9923=CARTESIAN_POINT('',(6.59756313292354,1.23743686707646,5.2));
#9924=CARTESIAN_POINT('',(6.59756313292354,1.23743686707646,4.1));
#9925=CARTESIAN_POINT('Origin',(6.76256313292354,1.23743686707646,5.2));
#9926=CARTESIAN_POINT('Origin',(6.76256313292354,1.23743686707646,4.1));
#9927=CARTESIAN_POINT('Origin',(9.23743686707646,1.23743686707646,4.1));
#9928=CARTESIAN_POINT('',(9.07243686707646,1.23743686707646,4.1));
#9929=CARTESIAN_POINT('Origin',(9.23743686707646,1.23743686707646,4.1));
#9930=CARTESIAN_POINT('',(9.07243686707646,1.23743686707646,5.2));
#9931=CARTESIAN_POINT('',(9.07243686707646,1.23743686707646,4.1));
#9932=CARTESIAN_POINT('Origin',(9.23743686707646,1.23743686707646,5.2));
#9933=CARTESIAN_POINT('Origin',(9.23743686707646,1.23743686707646,4.1));
#9934=CARTESIAN_POINT('Origin',(9.23743686707646,-1.23743686707646,4.1));
#9935=CARTESIAN_POINT('',(9.07243686707646,-1.23743686707646,4.1));
#9936=CARTESIAN_POINT('Origin',(9.23743686707646,-1.23743686707646,4.1));
#9937=CARTESIAN_POINT('',(9.07243686707646,-1.23743686707646,5.2));
#9938=CARTESIAN_POINT('',(9.07243686707646,-1.23743686707646,4.1));
#9939=CARTESIAN_POINT('Origin',(9.23743686707646,-1.23743686707646,5.2));
#9940=CARTESIAN_POINT('Origin',(9.23743686707646,-1.23743686707646,4.1));
#9941=CARTESIAN_POINT('Origin',(8.9,0.,1.4));
#9942=CARTESIAN_POINT('',(8.98888826466897,0.25,1.4));
#9943=CARTESIAN_POINT('',(9.02,1.2447490626287E-17,1.65));
#9944=CARTESIAN_POINT('Ctrl Pts',(8.98888826466897,0.25,1.4));
#9945=CARTESIAN_POINT('Ctrl Pts',(8.98888826466897,0.25,1.43153139415882));
#9946=CARTESIAN_POINT('Ctrl Pts',(8.99055337064667,0.243672048431404,1.46507214966317));
#9947=CARTESIAN_POINT('Ctrl Pts',(8.99649173729666,0.218119830014375,1.52662620974954));
#9948=CARTESIAN_POINT('Ctrl Pts',(9.00067109353237,0.198902128206072,1.5546512623872));
#9949=CARTESIAN_POINT('Ctrl Pts',(9.00845756932386,0.154654113568716,1.59889927702456));
#9950=CARTESIAN_POINT('Ctrl Pts',(9.01258144235289,0.126627870945253,1.61811920309393));
#9951=CARTESIAN_POINT('Ctrl Pts',(9.0183917429657,0.0650696003913631,1.64367304400768));
#9952=CARTESIAN_POINT('Ctrl Pts',(9.02,0.031527330883376,1.65));
#9953=CARTESIAN_POINT('Ctrl Pts',(9.02,3.46944695195361E-17,1.65));
#9954=CARTESIAN_POINT('Ctrl Pts',(9.02,3.46944695195361E-17,1.65));
#9955=CARTESIAN_POINT('Ctrl Pts',(9.02,-0.0315273308833759,1.65));
#9956=CARTESIAN_POINT('Ctrl Pts',(9.0183917429657,-0.065069600391363,1.64367304400768));
#9957=CARTESIAN_POINT('Ctrl Pts',(9.01258144235289,-0.126627870945253,1.61811920309393));
#9958=CARTESIAN_POINT('Ctrl Pts',(9.00845756932386,-0.154654113568716,1.59889927702456));
#9959=CARTESIAN_POINT('Ctrl Pts',(9.00067109353237,-0.198902128206072,1.5546512623872));
#9960=CARTESIAN_POINT('Ctrl Pts',(8.99649173729666,-0.218119830014375,1.52662620974954));
#9961=CARTESIAN_POINT('Ctrl Pts',(8.99055337064667,-0.243672048431404,1.46507214966317));
#9962=CARTESIAN_POINT('Ctrl Pts',(8.98888826466897,-0.25,1.43153139415882));
#9963=CARTESIAN_POINT('Ctrl Pts',(8.98888826466897,-0.25,1.36846860584118));
#9964=CARTESIAN_POINT('Ctrl Pts',(8.99055337064667,-0.243672048431404,1.33492785033683));
#9965=CARTESIAN_POINT('Ctrl Pts',(8.99649173729666,-0.218119830014375,1.27337379025046));
#9966=CARTESIAN_POINT('Ctrl Pts',(9.00067109353237,-0.198902128206072,1.2453487376128));
#9967=CARTESIAN_POINT('Ctrl Pts',(9.00845756932386,-0.154654113568716,1.20110072297544));
#9968=CARTESIAN_POINT('Ctrl Pts',(9.01258144235289,-0.126627870945253,1.18188079690607));
#9969=CARTESIAN_POINT('Ctrl Pts',(9.0183917429657,-0.0650696003913632,1.15632695599232));
#9970=CARTESIAN_POINT('Ctrl Pts',(9.02,-0.031527330883376,1.15));
#9971=CARTESIAN_POINT('Ctrl Pts',(9.02,0.0315273308833759,1.15));
#9972=CARTESIAN_POINT('Ctrl Pts',(9.0183917429657,0.065069600391363,1.15632695599232));
#9973=CARTESIAN_POINT('Ctrl Pts',(9.01258144235289,0.126627870945253,1.18188079690607));
#9974=CARTESIAN_POINT('Ctrl Pts',(9.00845756932386,0.154654113568716,1.20110072297544));
#9975=CARTESIAN_POINT('Ctrl Pts',(9.00067109353237,0.198902128206072,1.2453487376128));
#9976=CARTESIAN_POINT('Ctrl Pts',(8.99649173729666,0.218119830014375,1.27337379025046));
#9977=CARTESIAN_POINT('Ctrl Pts',(8.99055337064667,0.243672048431404,1.33492785033683));
#9978=CARTESIAN_POINT('Ctrl Pts',(8.98888826466897,0.25,1.36846860584118));
#9979=CARTESIAN_POINT('Ctrl Pts',(8.98888826466897,0.25,1.4));
#9980=CARTESIAN_POINT('',(11.,-3.06161699786838E-17,1.65));
#9981=CARTESIAN_POINT('',(8.9,-3.06161699786838E-17,1.65));
#9982=CARTESIAN_POINT('',(10.9895651857753,0.25,1.4));
#9983=CARTESIAN_POINT('Ctrl Pts',(10.9895651857753,0.25,1.4));
#9984=CARTESIAN_POINT('Ctrl Pts',(10.9895651857753,0.25,1.36859378633186));
#9985=CARTESIAN_POINT('Ctrl Pts',(10.9901110499518,0.24372047740942,1.33510417960069));
#9986=CARTESIAN_POINT('Ctrl Pts',(10.992081451651,0.218202539734559,1.27351367328886));
#9987=CARTESIAN_POINT('Ctrl Pts',(10.9934774080296,0.198964922639276,1.245411532046));
#9988=CARTESIAN_POINT('Ctrl Pts',(10.9960968651822,0.154588504271054,1.20103511367778));
#9989=CARTESIAN_POINT('Ctrl Pts',(10.997490703762,0.126486346986081,1.18179746841036));
#9990=CARTESIAN_POINT('Ctrl Pts',(10.9994562593684,0.064895787500922,1.15627950921557));
#9991=CARTESIAN_POINT('Ctrl Pts',(11.,0.0314061622633416,1.15));
#9992=CARTESIAN_POINT('Ctrl Pts',(11.,-0.0314061622633416,1.15));
#9993=CARTESIAN_POINT('Ctrl Pts',(10.9994562593684,-0.064895787500922,1.15627950921557));
#9994=CARTESIAN_POINT('Ctrl Pts',(10.997490703762,-0.126486346986081,1.18179746841036));
#9995=CARTESIAN_POINT('Ctrl Pts',(10.9960968651822,-0.154588504271054,1.20103511367778));
#9996=CARTESIAN_POINT('Ctrl Pts',(10.9934774080296,-0.198964922639276,1.245411532046));
#9997=CARTESIAN_POINT('Ctrl Pts',(10.992081451651,-0.218202539734559,1.27351367328886));
#9998=CARTESIAN_POINT('Ctrl Pts',(10.9901110499518,-0.24372047740942,1.33510417960069));
#9999=CARTESIAN_POINT('Ctrl Pts',(10.9895651857753,-0.25,1.36859378633186));
#10000=CARTESIAN_POINT('Ctrl Pts',(10.9895651857753,-0.25,1.43140621366814));
#10001=CARTESIAN_POINT('Ctrl Pts',(10.9901110499518,-0.24372047740942,1.4648958203993));
#10002=CARTESIAN_POINT('Ctrl Pts',(10.992081451651,-0.21820253973456,1.52648632671114));
#10003=CARTESIAN_POINT('Ctrl Pts',(10.9934774080296,-0.198964922639276,
1.554588467954));
#10004=CARTESIAN_POINT('Ctrl Pts',(10.9960968651822,-0.154588504271054,
1.59896488632222));
#10005=CARTESIAN_POINT('Ctrl Pts',(10.997490703762,-0.126486346986081,1.61820253158964));
#10006=CARTESIAN_POINT('Ctrl Pts',(10.9994562593684,-0.0648957875009221,
1.64372049078443));
#10007=CARTESIAN_POINT('Ctrl Pts',(11.,-0.0314061622633417,1.65));
#10008=CARTESIAN_POINT('Ctrl Pts',(11.,-4.85722573273506E-17,1.65));
#10009=CARTESIAN_POINT('Ctrl Pts',(11.,1.38777878078145E-17,1.65));
#10010=CARTESIAN_POINT('Ctrl Pts',(11.,0.0314061622633416,1.65));
#10011=CARTESIAN_POINT('Ctrl Pts',(10.9994562593684,0.064895787500922,1.64372049078443));
#10012=CARTESIAN_POINT('Ctrl Pts',(10.997490703762,0.126486346986081,1.61820253158964));
#10013=CARTESIAN_POINT('Ctrl Pts',(10.9960968651822,0.154588504271054,1.59896488632222));
#10014=CARTESIAN_POINT('Ctrl Pts',(10.9934774080296,0.198964922639276,1.554588467954));
#10015=CARTESIAN_POINT('Ctrl Pts',(10.992081451651,0.218202539734559,1.52648632671114));
#10016=CARTESIAN_POINT('Ctrl Pts',(10.9901110499518,0.24372047740942,1.46489582039931));
#10017=CARTESIAN_POINT('Ctrl Pts',(10.9895651857753,0.25,1.43140621366814));
#10018=CARTESIAN_POINT('Ctrl Pts',(10.9895651857753,0.25,1.4));
#10019=CARTESIAN_POINT('Origin',(6.23223304703363,-1.76776695296637,0.9));
#10020=CARTESIAN_POINT('',(5.95723304703363,-1.76776695296637,1.));
#10021=CARTESIAN_POINT('Origin',(6.23223304703363,-1.76776695296637,1.));
#10022=CARTESIAN_POINT('',(5.95723304703363,-1.76776695296637,0.9));
#10023=CARTESIAN_POINT('Origin',(6.23223304703363,1.76776695296637,0.9));
#10024=CARTESIAN_POINT('',(5.95723304703363,1.76776695296637,1.));
#10025=CARTESIAN_POINT('Origin',(6.23223304703363,1.76776695296637,1.));
#10026=CARTESIAN_POINT('',(5.95723304703363,1.76776695296637,0.9));
#10027=CARTESIAN_POINT('Origin',(9.76776695296637,1.76776695296637,0.9));
#10028=CARTESIAN_POINT('',(9.49276695296637,1.76776695296637,1.));
#10029=CARTESIAN_POINT('Origin',(9.76776695296637,1.76776695296637,1.));
#10030=CARTESIAN_POINT('',(9.49276695296637,1.76776695296637,0.9));
#10031=CARTESIAN_POINT('Origin',(9.76776695296637,-1.76776695296637,0.9));
#10032=CARTESIAN_POINT('',(9.49276695296637,-1.76776695296637,1.));
#10033=CARTESIAN_POINT('Origin',(9.76776695296637,-1.76776695296637,1.));
#10034=CARTESIAN_POINT('',(9.49276695296637,-1.76776695296637,0.9));
#10035=CARTESIAN_POINT('Origin',(8.,0.,3.05));
#10036=CARTESIAN_POINT('',(6.5,-1.83697019872103E-16,3.05));
#10037=CARTESIAN_POINT('Origin',(8.,0.,3.05));
#10038=CARTESIAN_POINT('',(6.5,1.83697019872103E-16,5.2));
#10039=CARTESIAN_POINT('',(6.5,-1.83697019872103E-16,3.05));
#10040=CARTESIAN_POINT('Origin',(8.,0.,5.2));
#10041=CARTESIAN_POINT('Origin',(8.,0.,3.05));
#10042=CARTESIAN_POINT('',(6.98,-1.2491397351303E-16,3.05));
#10043=CARTESIAN_POINT('Origin',(8.,0.,3.05));
#10044=CARTESIAN_POINT('Origin',(8.,0.,1.));
#10045=CARTESIAN_POINT('',(5.,-3.67394039744206E-16,1.));
#10046=CARTESIAN_POINT('',(5.,-3.67394039744206E-16,1.));
#10047=CARTESIAN_POINT('Origin',(8.,0.,1.));
#10048=CARTESIAN_POINT('Origin',(8.,0.,1.));
#10049=CARTESIAN_POINT('',(6.98,-1.2491397351303E-16,1.));
#10050=CARTESIAN_POINT('',(6.98,-1.2491397351303E-16,1.));
#10051=CARTESIAN_POINT('Origin',(8.,0.,1.));
#10052=CARTESIAN_POINT('Origin',(8.,0.,5.2));
#10053=CARTESIAN_POINT('Origin',(8.,0.,1.));
#11831=UNCERTAINTY_MEASURE_WITH_UNIT(LENGTH_MEASURE(0.001),#11917,
'DISTANCE_ACCURACY_VALUE',
'Maximum model space distance between geometric entities at asserted c
onnectivities');
#11869=UNCERTAINTY_MEASURE_WITH_UNIT(LENGTH_MEASURE(0.001),#11917,
'DISTANCE_ACCURACY_VALUE',
'Maximum model space distance between geometric entities at asserted c
onnectivities');
#11878=(
GEOMETRIC_REPRESENTATION_CONTEXT(3)
GLOBAL_UNCERTAINTY_ASSIGNED_CONTEXT((#11831))
GLOBAL_UNIT_ASSIGNED_CONTEXT((#11917,#11919,#11920))
REPRESENTATION_CONTEXT('','3D')
);
#11916=(
GEOMETRIC_REPRESENTATION_CONTEXT(3)
GLOBAL_UNCERTAINTY_ASSIGNED_CONTEXT((#11869))
GLOBAL_UNIT_ASSIGNED_CONTEXT((#11917,#11919,#11920))
REPRESENTATION_CONTEXT('','3D')
);
#11917=(
LENGTH_UNIT()
NAMED_UNIT(*)
SI_UNIT(.CENTI.,.METRE.)
);
#11919=(
NAMED_UNIT(*)
PLANE_ANGLE_UNIT()
SI_UNIT($,.RADIAN.)
);
#11920=(
NAMED_UNIT(*)
SI_UNIT($,.STERADIAN.)
SOLID_ANGLE_UNIT()
);
#11929=SHAPE_DEFINITION_REPRESENTATION(#11975,#12087);
#11975=PRODUCT_DEFINITION_SHAPE('',$,#12134);
#12087=SHAPE_REPRESENTATION('',(#6710),#11878);
#12125=PRODUCT_DEFINITION_CONTEXT('part definition',#12265,'design');
#12134=PRODUCT_DEFINITION('Output pedestal','Output pedestal',#12180,#12125);
#12180=PRODUCT_DEFINITION_FORMATION('',$,#12275);
#12265=APPLICATION_CONTEXT(
'Core Data for Automotive Mechanical Design Process');
#12266=PRODUCT_CONTEXT('part definition',#12265,'mechanical');
#12275=PRODUCT('Output pedestal','Output pedestal','Output pedestal',(#12266));
#12362=COLOUR_RGB('Sky Blue',0.24,0.69,0.87);
#12363=FILL_AREA_STYLE_COLOUR('',#12362);
#12364=FILL_AREA_STYLE('',(#12363));
#12365=SURFACE_STYLE_FILL_AREA(#12364);
#12366=SURFACE_SIDE_STYLE('',(#12365));
#12367=SURFACE_STYLE_USAGE(.BOTH.,#12366);
#12368=PRESENTATION_STYLE_ASSIGNMENT((#12367));
ENDSEC;
END-ISO-10303-21;
